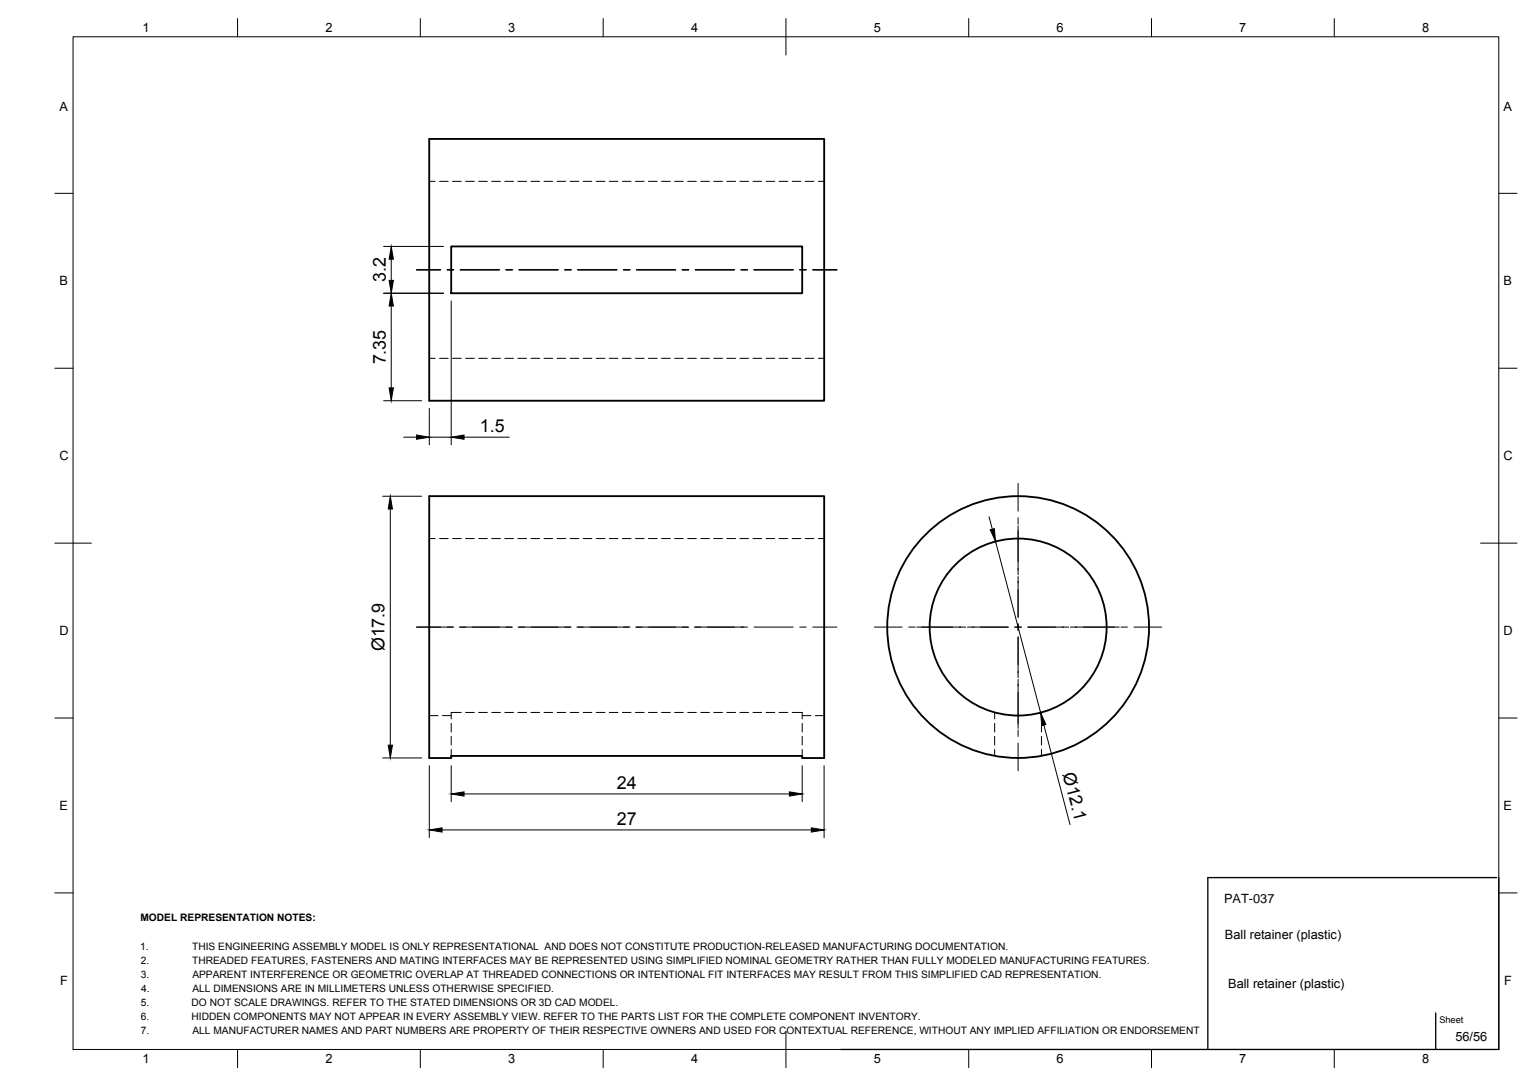
ISO-10303-21;
HEADER;
/* Generated by software containing ST-Developer
 * from STEP Tools, Inc. (www.steptools.com) 
 */

FILE_DESCRIPTION(
/* description */ ('Flywheel Crank-Slider'),
/* implementation_level */ '2;1');

FILE_NAME(
/* name */ 'Ball retainer (plastic).step',
/* time_stamp */ '2026-10-28T03:23:13-07:00',
/* author */ (''),
/* organization */ (''),
/* preprocessor_version */ 'ST-DEVELOPER v20.2',
/* originating_system */ 'Autodesk Translation Framework v15.17.0.0',
/* authorisation */ '');

FILE_SCHEMA (('AUTOMOTIVE_DESIGN { 1 0 10303 214 3 1 1 }'));
ENDSEC;

DATA;
#10=MECHANICAL_DESIGN_GEOMETRIC_PRESENTATION_REPRESENTATION('',(#727),#17322);
#614=SHAPE_REPRESENTATION_RELATIONSHIP('SRR','None',#17616,#666);
#666=ADVANCED_BREP_SHAPE_REPRESENTATION('',(#784),#17320);
#727=STYLED_ITEM('',(#17924),#784);
#784=MANIFOLD_SOLID_BREP('Body1',#9109);
#1006=FACE_BOUND('',#2592,.T.);
#1007=FACE_BOUND('',#2594,.T.);
#1008=FACE_BOUND('',#2596,.T.);
#1009=FACE_BOUND('',#2598,.T.);
#1303=PLANE('',#10693);
#1304=PLANE('',#10696);
#1305=PLANE('',#10697);
#1306=PLANE('',#10700);
#1307=PLANE('',#10701);
#1308=PLANE('',#10706);
#1831=FACE_OUTER_BOUND('',#2587,.T.);
#1832=FACE_OUTER_BOUND('',#2588,.T.);
#1833=FACE_OUTER_BOUND('',#2589,.T.);
#1834=FACE_OUTER_BOUND('',#2590,.T.);
#1835=FACE_OUTER_BOUND('',#2591,.T.);
#1836=FACE_OUTER_BOUND('',#2593,.T.);
#1837=FACE_OUTER_BOUND('',#2595,.T.);
#1838=FACE_OUTER_BOUND('',#2597,.T.);
#2587=EDGE_LOOP('',(#8234,#8235,#8236,#8237));
#2588=EDGE_LOOP('',(#8238,#8239,#8240,#8241));
#2589=EDGE_LOOP('',(#8242,#8243,#8244,#8245));
#2590=EDGE_LOOP('',(#8246,#8247,#8248,#8249));
#2591=EDGE_LOOP('',(#8250));
#2592=EDGE_LOOP('',(#8251));
#2593=EDGE_LOOP('',(#8252,#8253,#8254,#8255));
#2594=EDGE_LOOP('',(#8256,#8257,#8258,#8259));
#2595=EDGE_LOOP('',(#8260));
#2596=EDGE_LOOP('',(#8261));
#2597=EDGE_LOOP('',(#8262,#8263,#8264,#8265));
#2598=EDGE_LOOP('',(#8266,#8267,#8268,#8269));
#3194=LINE('',#17005,#3805);
#3195=LINE('',#17008,#3806);
#3196=LINE('',#17011,#3807);
#3197=LINE('',#17013,#3808);
#3198=LINE('',#17014,#3809);
#3199=LINE('',#17020,#3810);
#3200=LINE('',#17022,#3811);
#3201=LINE('',#17023,#3812);
#3202=LINE('',#17032,#3813);
#3203=LINE('',#17037,#3814);
#3805=VECTOR('',#13428,1.);
#3806=VECTOR('',#13431,1.);
#3807=VECTOR('',#13434,1.);
#3808=VECTOR('',#13435,1.);
#3809=VECTOR('',#13436,1.);
#3810=VECTOR('',#13443,1.);
#3811=VECTOR('',#13446,1.);
#3812=VECTOR('',#13447,1.);
#3813=VECTOR('',#13458,0.895);
#3814=VECTOR('',#13465,0.605);
#4262=CIRCLE('',#10694,0.895);
#4263=CIRCLE('',#10695,0.605);
#4264=CIRCLE('',#10698,0.895);
#4265=CIRCLE('',#10699,0.605);
#4266=CIRCLE('',#10702,0.895);
#4267=CIRCLE('',#10703,0.605);
#4268=CIRCLE('',#10705,0.895);
#4269=CIRCLE('',#10707,0.605);
#4987=VERTEX_POINT('',#17001);
#4988=VERTEX_POINT('',#17002);
#4989=VERTEX_POINT('',#17004);
#4990=VERTEX_POINT('',#17006);
#4991=VERTEX_POINT('',#17010);
#4992=VERTEX_POINT('',#17012);
#4993=VERTEX_POINT('',#17016);
#4994=VERTEX_POINT('',#17018);
#4995=VERTEX_POINT('',#17025);
#4996=VERTEX_POINT('',#17027);
#4997=VERTEX_POINT('',#17030);
#4998=VERTEX_POINT('',#17034);
#6074=EDGE_CURVE('',#4987,#4988,#4262,.T.);
#6075=EDGE_CURVE('',#4989,#4987,#3194,.T.);
#6076=EDGE_CURVE('',#4990,#4989,#4263,.T.);
#6077=EDGE_CURVE('',#4988,#4990,#3195,.T.);
#6078=EDGE_CURVE('',#4988,#4991,#3196,.T.);
#6079=EDGE_CURVE('',#4992,#4990,#3197,.T.);
#6080=EDGE_CURVE('',#4992,#4991,#3198,.T.);
#6081=EDGE_CURVE('',#4991,#4993,#4264,.T.);
#6082=EDGE_CURVE('',#4994,#4992,#4265,.T.);
#6083=EDGE_CURVE('',#4993,#4994,#3199,.T.);
#6084=EDGE_CURVE('',#4993,#4987,#3200,.T.);
#6085=EDGE_CURVE('',#4989,#4994,#3201,.T.);
#6086=EDGE_CURVE('',#4995,#4995,#4266,.T.);
#6087=EDGE_CURVE('',#4996,#4996,#4267,.T.);
#6088=EDGE_CURVE('',#4997,#4997,#4268,.T.);
#6089=EDGE_CURVE('',#4997,#4995,#3202,.T.);
#6090=EDGE_CURVE('',#4998,#4998,#4269,.T.);
#6091=EDGE_CURVE('',#4998,#4996,#3203,.T.);
#8234=ORIENTED_EDGE('',*,*,#6074,.F.);
#8235=ORIENTED_EDGE('',*,*,#6075,.F.);
#8236=ORIENTED_EDGE('',*,*,#6076,.F.);
#8237=ORIENTED_EDGE('',*,*,#6077,.F.);
#8238=ORIENTED_EDGE('',*,*,#6078,.F.);
#8239=ORIENTED_EDGE('',*,*,#6077,.T.);
#8240=ORIENTED_EDGE('',*,*,#6079,.F.);
#8241=ORIENTED_EDGE('',*,*,#6080,.T.);
#8242=ORIENTED_EDGE('',*,*,#6081,.F.);
#8243=ORIENTED_EDGE('',*,*,#6080,.F.);
#8244=ORIENTED_EDGE('',*,*,#6082,.F.);
#8245=ORIENTED_EDGE('',*,*,#6083,.F.);
#8246=ORIENTED_EDGE('',*,*,#6084,.F.);
#8247=ORIENTED_EDGE('',*,*,#6083,.T.);
#8248=ORIENTED_EDGE('',*,*,#6085,.F.);
#8249=ORIENTED_EDGE('',*,*,#6075,.T.);
#8250=ORIENTED_EDGE('',*,*,#6086,.F.);
#8251=ORIENTED_EDGE('',*,*,#6087,.T.);
#8252=ORIENTED_EDGE('',*,*,#6088,.F.);
#8253=ORIENTED_EDGE('',*,*,#6089,.T.);
#8254=ORIENTED_EDGE('',*,*,#6086,.T.);
#8255=ORIENTED_EDGE('',*,*,#6089,.F.);
#8256=ORIENTED_EDGE('',*,*,#6081,.T.);
#8257=ORIENTED_EDGE('',*,*,#6084,.T.);
#8258=ORIENTED_EDGE('',*,*,#6074,.T.);
#8259=ORIENTED_EDGE('',*,*,#6078,.T.);
#8260=ORIENTED_EDGE('',*,*,#6088,.T.);
#8261=ORIENTED_EDGE('',*,*,#6090,.F.);
#8262=ORIENTED_EDGE('',*,*,#6090,.T.);
#8263=ORIENTED_EDGE('',*,*,#6091,.T.);
#8264=ORIENTED_EDGE('',*,*,#6087,.F.);
#8265=ORIENTED_EDGE('',*,*,#6091,.F.);
#8266=ORIENTED_EDGE('',*,*,#6082,.T.);
#8267=ORIENTED_EDGE('',*,*,#6079,.T.);
#8268=ORIENTED_EDGE('',*,*,#6076,.T.);
#8269=ORIENTED_EDGE('',*,*,#6085,.T.);
#8507=CYLINDRICAL_SURFACE('',#10704,0.895);
#8508=CYLINDRICAL_SURFACE('',#10708,0.605);
#9022=ADVANCED_FACE('',(#1831),#1303,.F.);
#9023=ADVANCED_FACE('',(#1832),#1304,.F.);
#9024=ADVANCED_FACE('',(#1833),#1305,.F.);
#9025=ADVANCED_FACE('',(#1834),#1306,.F.);
#9026=ADVANCED_FACE('',(#1835,#1006),#1307,.T.);
#9027=ADVANCED_FACE('',(#1836,#1007),#8507,.T.);
#9028=ADVANCED_FACE('',(#1837,#1008),#1308,.T.);
#9029=ADVANCED_FACE('',(#1838,#1009),#8508,.F.);
#9109=CLOSED_SHELL('',(#9022,#9023,#9024,#9025,#9026,#9027,#9028,#9029));
#10692=AXIS2_PLACEMENT_3D('',#16999,#13422,#13423);
#10693=AXIS2_PLACEMENT_3D('',#17000,#13424,#13425);
#10694=AXIS2_PLACEMENT_3D('',#17003,#13426,#13427);
#10695=AXIS2_PLACEMENT_3D('',#17007,#13429,#13430);
#10696=AXIS2_PLACEMENT_3D('',#17009,#13432,#13433);
#10697=AXIS2_PLACEMENT_3D('',#17015,#13437,#13438);
#10698=AXIS2_PLACEMENT_3D('',#17017,#13439,#13440);
#10699=AXIS2_PLACEMENT_3D('',#17019,#13441,#13442);
#10700=AXIS2_PLACEMENT_3D('',#17021,#13444,#13445);
#10701=AXIS2_PLACEMENT_3D('',#17024,#13448,#13449);
#10702=AXIS2_PLACEMENT_3D('',#17026,#13450,#13451);
#10703=AXIS2_PLACEMENT_3D('',#17028,#13452,#13453);
#10704=AXIS2_PLACEMENT_3D('',#17029,#13454,#13455);
#10705=AXIS2_PLACEMENT_3D('',#17031,#13456,#13457);
#10706=AXIS2_PLACEMENT_3D('',#17033,#13459,#13460);
#10707=AXIS2_PLACEMENT_3D('',#17035,#13461,#13462);
#10708=AXIS2_PLACEMENT_3D('',#17036,#13463,#13464);
#13422=DIRECTION('axis',(0.,0.,1.));
#13423=DIRECTION('refdir',(1.,0.,0.));
#13424=DIRECTION('center_axis',(0.,1.,0.));
#13425=DIRECTION('ref_axis',(0.,0.,1.));
#13426=DIRECTION('center_axis',(0.,1.,0.));
#13427=DIRECTION('ref_axis',(1.,0.,0.));
#13428=DIRECTION('',(1.,0.,0.));
#13429=DIRECTION('center_axis',(0.,-1.,0.));
#13430=DIRECTION('ref_axis',(1.,0.,0.));
#13431=DIRECTION('',(-1.,0.,0.));
#13432=DIRECTION('center_axis',(0.,0.,-1.));
#13433=DIRECTION('ref_axis',(-1.,0.,0.));
#13434=DIRECTION('',(0.,-1.,0.));
#13435=DIRECTION('',(0.,1.,0.));
#13436=DIRECTION('',(1.,0.,0.));
#13437=DIRECTION('center_axis',(0.,-1.,0.));
#13438=DIRECTION('ref_axis',(0.,0.,-1.));
#13439=DIRECTION('center_axis',(0.,-1.,0.));
#13440=DIRECTION('ref_axis',(1.,0.,0.));
#13441=DIRECTION('center_axis',(0.,1.,0.));
#13442=DIRECTION('ref_axis',(1.,0.,0.));
#13443=DIRECTION('',(-1.,0.,0.));
#13444=DIRECTION('center_axis',(0.,0.,1.));
#13445=DIRECTION('ref_axis',(1.,0.,0.));
#13446=DIRECTION('',(0.,1.,0.));
#13447=DIRECTION('',(0.,-1.,0.));
#13448=DIRECTION('center_axis',(0.,1.,0.));
#13449=DIRECTION('ref_axis',(0.,0.,1.));
#13450=DIRECTION('center_axis',(0.,-1.,0.));
#13451=DIRECTION('ref_axis',(1.,0.,0.));
#13452=DIRECTION('center_axis',(0.,-1.,0.));
#13453=DIRECTION('ref_axis',(1.,0.,0.));
#13454=DIRECTION('center_axis',(0.,-1.,0.));
#13455=DIRECTION('ref_axis',(1.,0.,0.));
#13456=DIRECTION('center_axis',(0.,-1.,0.));
#13457=DIRECTION('ref_axis',(1.,0.,0.));
#13458=DIRECTION('',(0.,1.,0.));
#13459=DIRECTION('center_axis',(0.,-1.,0.));
#13460=DIRECTION('ref_axis',(0.,0.,-1.));
#13461=DIRECTION('center_axis',(0.,-1.,0.));
#13462=DIRECTION('ref_axis',(1.,0.,0.));
#13463=DIRECTION('center_axis',(0.,-1.,0.));
#13464=DIRECTION('ref_axis',(1.,0.,0.));
#13465=DIRECTION('',(0.,1.,0.));
#16999=CARTESIAN_POINT('',(0.,0.,0.));
#17000=CARTESIAN_POINT('Origin',(0.75,1.2,0.));
#17001=CARTESIAN_POINT('',(0.880582193778639,1.2,0.16));
#17002=CARTESIAN_POINT('',(0.880582193778639,1.2,-0.16));
#17003=CARTESIAN_POINT('Origin',(0.,1.2,0.));
#17004=CARTESIAN_POINT('',(0.583459510163302,1.2,0.16));
#17005=CARTESIAN_POINT('',(0.57,1.2,0.16));
#17006=CARTESIAN_POINT('',(0.583459510163302,1.2,-0.16));
#17007=CARTESIAN_POINT('Origin',(0.,1.2,0.));
#17008=CARTESIAN_POINT('',(0.93,1.2,-0.16));
#17009=CARTESIAN_POINT('Origin',(0.93,0.,-0.16));
#17010=CARTESIAN_POINT('',(0.880582193778639,-1.2,-0.16));
#17011=CARTESIAN_POINT('',(0.880582193778639,0.,-0.16));
#17012=CARTESIAN_POINT('',(0.583459510163302,-1.2,-0.16));
#17013=CARTESIAN_POINT('',(0.583459510163302,0.,-0.16));
#17014=CARTESIAN_POINT('',(0.93,-1.2,-0.16));
#17015=CARTESIAN_POINT('Origin',(0.75,-1.2,0.));
#17016=CARTESIAN_POINT('',(0.880582193778639,-1.2,0.16));
#17017=CARTESIAN_POINT('Origin',(0.,-1.2,0.));
#17018=CARTESIAN_POINT('',(0.583459510163302,-1.2,0.16));
#17019=CARTESIAN_POINT('Origin',(0.,-1.2,0.));
#17020=CARTESIAN_POINT('',(0.57,-1.2,0.16));
#17021=CARTESIAN_POINT('Origin',(0.57,0.,0.16));
#17022=CARTESIAN_POINT('',(0.880582193778639,0.,0.16));
#17023=CARTESIAN_POINT('',(0.583459510163302,0.,0.16));
#17024=CARTESIAN_POINT('Origin',(0.895,1.35,0.));
#17025=CARTESIAN_POINT('',(-0.895,1.35,-1.09605888523688E-16));
#17026=CARTESIAN_POINT('Origin',(0.,1.35,0.));
#17027=CARTESIAN_POINT('',(-0.605,1.35,-7.40911313484149E-17));
#17028=CARTESIAN_POINT('Origin',(0.,1.35,0.));
#17029=CARTESIAN_POINT('Origin',(0.,0.,0.));
#17030=CARTESIAN_POINT('',(-0.895,-1.35,-1.09605888523688E-16));
#17031=CARTESIAN_POINT('Origin',(0.,-1.35,0.));
#17032=CARTESIAN_POINT('',(-0.895,0.,-1.09605888523688E-16));
#17033=CARTESIAN_POINT('Origin',(0.605,-1.35,0.));
#17034=CARTESIAN_POINT('',(-0.605,-1.35,-7.40911313484149E-17));
#17035=CARTESIAN_POINT('Origin',(0.,-1.35,0.));
#17036=CARTESIAN_POINT('Origin',(0.,0.,0.));
#17037=CARTESIAN_POINT('',(-0.605,0.,-7.40911313484149E-17));
#17259=UNCERTAINTY_MEASURE_WITH_UNIT(LENGTH_MEASURE(0.001),#17323,
'DISTANCE_ACCURACY_VALUE',
'Maximum model space distance between geometric entities at asserted c
onnectivities');
#17261=UNCERTAINTY_MEASURE_WITH_UNIT(LENGTH_MEASURE(0.001),#17323,
'DISTANCE_ACCURACY_VALUE',
'Maximum model space distance between geometric entities at asserted c
onnectivities');
#17320=(
GEOMETRIC_REPRESENTATION_CONTEXT(3)
GLOBAL_UNCERTAINTY_ASSIGNED_CONTEXT((#17259))
GLOBAL_UNIT_ASSIGNED_CONTEXT((#17323,#17325,#17326))
REPRESENTATION_CONTEXT('','3D')
);
#17322=(
GEOMETRIC_REPRESENTATION_CONTEXT(3)
GLOBAL_UNCERTAINTY_ASSIGNED_CONTEXT((#17261))
GLOBAL_UNIT_ASSIGNED_CONTEXT((#17323,#17325,#17326))
REPRESENTATION_CONTEXT('','3D')
);
#17323=(
LENGTH_UNIT()
NAMED_UNIT(*)
SI_UNIT(.CENTI.,.METRE.)
);
#17325=(
NAMED_UNIT(*)
PLANE_ANGLE_UNIT()
SI_UNIT($,.RADIAN.)
);
#17326=(
NAMED_UNIT(*)
SI_UNIT($,.STERADIAN.)
SOLID_ANGLE_UNIT()
);
#17385=SHAPE_DEFINITION_REPRESENTATION(#17459,#17616);
#17459=PRODUCT_DEFINITION_SHAPE('',$,#17677);
#17616=SHAPE_REPRESENTATION('',(#10692),#17320);
#17618=PRODUCT_DEFINITION_CONTEXT('part definition',#17800,'design');
#17677=PRODUCT_DEFINITION('Ball retainer (plastic)',
'Ball retainer (plastic)',#17737,#17618);
#17737=PRODUCT_DEFINITION_FORMATION('',$,#17860);
#17800=APPLICATION_CONTEXT(
'Core Data for Automotive Mechanical Design Process');
#17801=PRODUCT_CONTEXT('part definition',#17800,'mechanical');
#17860=PRODUCT('Ball retainer (plastic)','Ball retainer (plastic)',
'Ball retainer (plastic)',(#17801));
#17918=COLOUR_RGB('Sky Blue',0.24,0.69,0.87);
#17919=FILL_AREA_STYLE_COLOUR('',#17918);
#17920=FILL_AREA_STYLE('',(#17919));
#17921=SURFACE_STYLE_FILL_AREA(#17920);
#17922=SURFACE_SIDE_STYLE('',(#17921));
#17923=SURFACE_STYLE_USAGE(.BOTH.,#17922);
#17924=PRESENTATION_STYLE_ASSIGNMENT((#17923));
ENDSEC;
END-ISO-10303-21;
